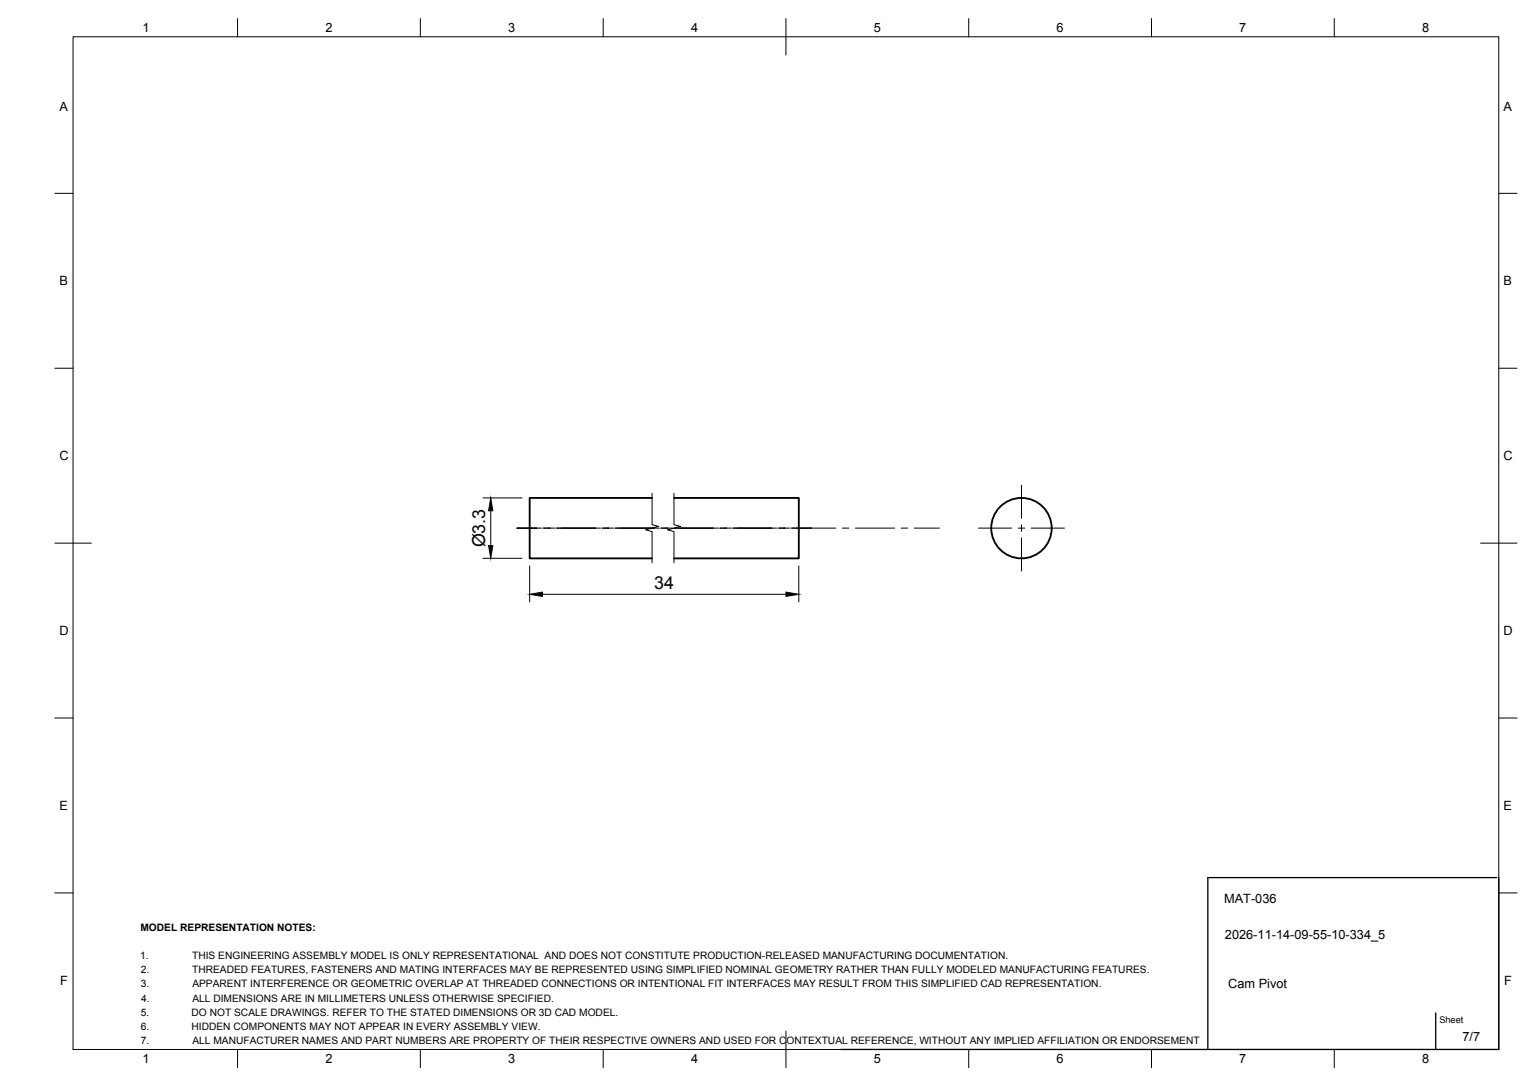
ISO-10303-21;
HEADER;
/* Generated by software containing ST-Developer
 * from STEP Tools, Inc. (www.steptools.com) 
 */

FILE_DESCRIPTION(
/* description */ (''),
/* implementation_level */ '2;1');

FILE_NAME(
/* name */ 'Cam Pivot.step',
/* time_stamp */ '2026-11-14T09:55:16-08:00',
/* author */ (''),
/* organization */ (''),
/* preprocessor_version */ 'ST-DEVELOPER v20.2',
/* originating_system */ 'Autodesk Translation Framework v15.17.0.0',
/* authorisation */ '');

FILE_SCHEMA (('AUTOMOTIVE_DESIGN { 1 0 10303 214 3 1 1 }'));
ENDSEC;

DATA;
#10=MECHANICAL_DESIGN_GEOMETRIC_PRESENTATION_REPRESENTATION('',(#63),#170250);
#49=SHAPE_REPRESENTATION_RELATIONSHIP('SRR','None',#170281,#55);
#55=ADVANCED_BREP_SHAPE_REPRESENTATION('',(#69),#170249);
#63=STYLED_ITEM('',(#170315),#69);
#69=MANIFOLD_SOLID_BREP('Body1',#71403);
#110=PLANE('',#77755);
#111=PLANE('',#77756);
#5382=CYLINDRICAL_SURFACE('',#77752,1.65);
#10645=FACE_OUTER_BOUND('',#15926,.T.);
#10646=FACE_OUTER_BOUND('',#15927,.T.);
#10647=FACE_OUTER_BOUND('',#15928,.T.);
#15926=EDGE_LOOP('',(#65998,#65999,#66000,#66001));
#15927=EDGE_LOOP('',(#66002));
#15928=EDGE_LOOP('',(#66003));
#21044=CIRCLE('',#77753,1.65);
#21045=CIRCLE('',#77754,1.65);
#26444=LINE('',#170225,#28532);
#28532=VECTOR('',#92416,1.65);
#33962=VERTEX_POINT('',#170222);
#33963=VERTEX_POINT('',#170224);
#44643=EDGE_CURVE('',#33962,#33962,#21044,.T.);
#44644=EDGE_CURVE('',#33962,#33963,#26444,.T.);
#44645=EDGE_CURVE('',#33963,#33963,#21045,.T.);
#65998=ORIENTED_EDGE('',*,*,#44643,.F.);
#65999=ORIENTED_EDGE('',*,*,#44644,.T.);
#66000=ORIENTED_EDGE('',*,*,#44645,.F.);
#66001=ORIENTED_EDGE('',*,*,#44644,.F.);
#66002=ORIENTED_EDGE('',*,*,#44643,.T.);
#66003=ORIENTED_EDGE('',*,*,#44645,.T.);
#71395=ADVANCED_FACE('',(#10645),#5382,.T.);
#71396=ADVANCED_FACE('',(#10646),#110,.T.);
#71397=ADVANCED_FACE('',(#10647),#111,.F.);
#71403=CLOSED_SHELL('',(#71395,#71396,#71397));
#77751=AXIS2_PLACEMENT_3D('',#170220,#92410,#92411);
#77752=AXIS2_PLACEMENT_3D('',#170221,#92412,#92413);
#77753=AXIS2_PLACEMENT_3D('',#170223,#92414,#92415);
#77754=AXIS2_PLACEMENT_3D('',#170226,#92417,#92418);
#77755=AXIS2_PLACEMENT_3D('',#170227,#92419,#92420);
#77756=AXIS2_PLACEMENT_3D('',#170228,#92421,#92422);
#92410=DIRECTION('axis',(0.,0.,1.));
#92411=DIRECTION('refdir',(1.,0.,0.));
#92412=DIRECTION('center_axis',(7.17905020382051E-15,1.,7.17905020446514E-15));
#92413=DIRECTION('ref_axis',(8.84265355443813E-30,-7.17905020446514E-15,
1.));
#92414=DIRECTION('center_axis',(7.17905020382051E-15,1.,7.17905020446514E-15));
#92415=DIRECTION('ref_axis',(1.09063096933567E-44,-7.17905020446514E-15,
1.));
#92416=DIRECTION('',(-7.17905020382051E-15,-1.,-7.17905020446514E-15));
#92417=DIRECTION('center_axis',(-7.17905020382051E-15,-1.,-7.17905020446514E-15));
#92418=DIRECTION('ref_axis',(8.84265355443813E-30,-7.17905020446514E-15,
1.));
#92419=DIRECTION('center_axis',(0.,1.,0.));
#92420=DIRECTION('ref_axis',(1.,0.,0.));
#92421=DIRECTION('center_axis',(0.,1.,0.));
#92422=DIRECTION('ref_axis',(1.,0.,0.));
#170220=CARTESIAN_POINT('',(0.,0.,0.));
#170221=CARTESIAN_POINT('Origin',(-2.37021530919249E-15,-34.,-1.9011994468366E-15));
#170222=CARTESIAN_POINT('',(2.41515424898845E-13,0.,-1.64999999999976));
#170223=CARTESIAN_POINT('Origin',(2.41717491620705E-13,-1.38777878078145E-14,
2.42186507504978E-13));
#170224=CARTESIAN_POINT('',(-2.57228203105183E-15,-34.,-1.65));
#170225=CARTESIAN_POINT('',(-2.57228203105182E-15,-34.,-1.65));
#170226=CARTESIAN_POINT('Origin',(-2.37021530919251E-15,-34.,-1.90119944683662E-15));
#170227=CARTESIAN_POINT('Origin',(-1.6698,0.,-1.6698));
#170228=CARTESIAN_POINT('Origin',(-1.6698,-34.,-1.6698));
#170241=UNCERTAINTY_MEASURE_WITH_UNIT(LENGTH_MEASURE(0.01),#170251,
'DISTANCE_ACCURACY_VALUE',
'Maximum model space distance between geometric entities at asserted c
onnectivities');
#170242=UNCERTAINTY_MEASURE_WITH_UNIT(LENGTH_MEASURE(0.01),#170251,
'DISTANCE_ACCURACY_VALUE',
'Maximum model space distance between geometric entities at asserted c
onnectivities');
#170249=(
GEOMETRIC_REPRESENTATION_CONTEXT(3)
GLOBAL_UNCERTAINTY_ASSIGNED_CONTEXT((#170241))
GLOBAL_UNIT_ASSIGNED_CONTEXT((#170251,#170253,#170254))
REPRESENTATION_CONTEXT('','3D')
);
#170250=(
GEOMETRIC_REPRESENTATION_CONTEXT(3)
GLOBAL_UNCERTAINTY_ASSIGNED_CONTEXT((#170242))
GLOBAL_UNIT_ASSIGNED_CONTEXT((#170251,#170253,#170254))
REPRESENTATION_CONTEXT('','3D')
);
#170251=(
LENGTH_UNIT()
NAMED_UNIT(*)
SI_UNIT(.MILLI.,.METRE.)
);
#170253=(
NAMED_UNIT(*)
PLANE_ANGLE_UNIT()
SI_UNIT($,.RADIAN.)
);
#170254=(
NAMED_UNIT(*)
SI_UNIT($,.STERADIAN.)
SOLID_ANGLE_UNIT()
);
#170261=SHAPE_DEFINITION_REPRESENTATION(#170268,#170281);
#170268=PRODUCT_DEFINITION_SHAPE('',$,#170289);
#170281=SHAPE_REPRESENTATION('',(#77751),#170249);
#170282=PRODUCT_DEFINITION_CONTEXT('part definition',#170305,'design');
#170289=PRODUCT_DEFINITION('2026-11-14-09-55-10-334_5','Cam Pivot',#170296,
#170282);
#170296=PRODUCT_DEFINITION_FORMATION('',$,#170313);
#170305=APPLICATION_CONTEXT(
'Core Data for Automotive Mechanical Design Process');
#170306=PRODUCT_CONTEXT('part definition',#170305,'mechanical');
#170313=PRODUCT('2026-11-14-09-55-10-334_5','Cam Pivot',$,(#170306));
#170315=PRESENTATION_STYLE_ASSIGNMENT((#170319));
#170319=SURFACE_STYLE_USAGE(.BOTH.,#170323);
#170323=SURFACE_SIDE_STYLE('',(#170327));
#170327=SURFACE_STYLE_FILL_AREA(#170331);
#170331=FILL_AREA_STYLE('Opaque(227,224,212)',(#170335));
#170335=FILL_AREA_STYLE_COLOUR('Opaque(227,224,212)',#170339);
#170339=COLOUR_RGB('Opaque(227,224,212)',0.890196078431372,0.87843137254902,
0.831372549019608);
ENDSEC;
END-ISO-10303-21;
